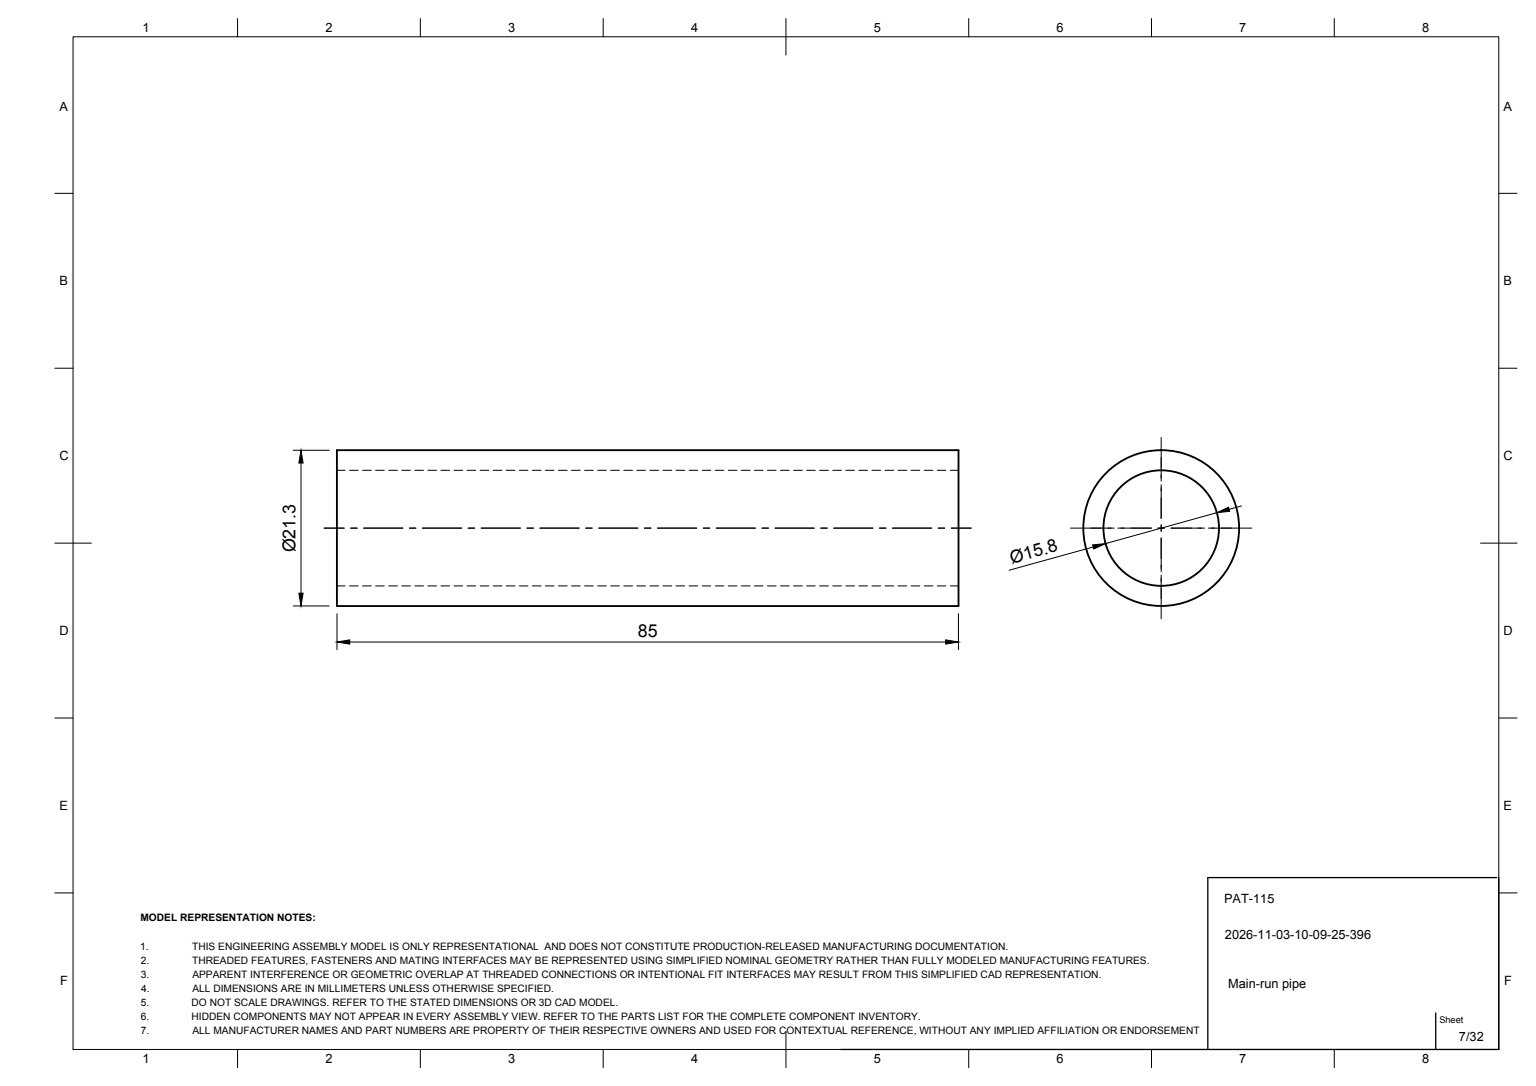
ISO-10303-21;
HEADER;
/* Generated by software containing ST-Developer
 * from STEP Tools, Inc. (www.steptools.com) 
 */

FILE_DESCRIPTION(
/* description */ ('Union bypass pipe loop'),
/* implementation_level */ '2;1');

FILE_NAME(
/* name */ 'Main-run pipe.step',
/* time_stamp */ '2026-10-27T21:00:29-07:00',
/* author */ (''),
/* organization */ (''),
/* preprocessor_version */ 'ST-DEVELOPER v20.2',
/* originating_system */ 'Autodesk Translation Framework v15.17.0.0',
/* authorisation */ '');

FILE_SCHEMA (('AUTOMOTIVE_DESIGN { 1 0 10303 214 3 1 1 }'));
ENDSEC;

DATA;
#10=MECHANICAL_DESIGN_GEOMETRIC_PRESENTATION_REPRESENTATION('',(#461),#10095);
#397=SHAPE_REPRESENTATION_RELATIONSHIP('SRR','None',#10266,#429);
#429=ADVANCED_BREP_SHAPE_REPRESENTATION('',(#491),#10078);
#461=STYLED_ITEM('',(#10486),#491);
#491=MANIFOLD_SOLID_BREP('Body1',#5534);
#582=FACE_BOUND('',#1413,.T.);
#583=FACE_BOUND('',#1415,.T.);
#732=PLANE('',#6291);
#733=PLANE('',#6292);
#1007=FACE_OUTER_BOUND('',#1410,.T.);
#1008=FACE_OUTER_BOUND('',#1411,.T.);
#1009=FACE_OUTER_BOUND('',#1412,.T.);
#1010=FACE_OUTER_BOUND('',#1414,.T.);
#1410=EDGE_LOOP('',(#4440,#4441,#4442,#4443));
#1411=EDGE_LOOP('',(#4444,#4445,#4446,#4447));
#1412=EDGE_LOOP('',(#4448));
#1413=EDGE_LOOP('',(#4449));
#1414=EDGE_LOOP('',(#4450));
#1415=EDGE_LOOP('',(#4451));
#1809=LINE('',#9257,#2185);
#1810=LINE('',#9263,#2186);
#2185=VECTOR('',#7569,0.79);
#2186=VECTOR('',#7576,1.065);
#2514=CIRCLE('',#6286,0.79);
#2515=CIRCLE('',#6287,0.79);
#2516=CIRCLE('',#6289,1.065);
#2517=CIRCLE('',#6290,1.065);
#2858=VERTEX_POINT('',#9254);
#2859=VERTEX_POINT('',#9256);
#2860=VERTEX_POINT('',#9260);
#2861=VERTEX_POINT('',#9262);
#3418=EDGE_CURVE('',#2858,#2858,#2514,.T.);
#3419=EDGE_CURVE('',#2858,#2859,#1809,.T.);
#3420=EDGE_CURVE('',#2859,#2859,#2515,.T.);
#3421=EDGE_CURVE('',#2860,#2860,#2516,.T.);
#3422=EDGE_CURVE('',#2860,#2861,#1810,.T.);
#3423=EDGE_CURVE('',#2861,#2861,#2517,.T.);
#4440=ORIENTED_EDGE('',*,*,#3418,.F.);
#4441=ORIENTED_EDGE('',*,*,#3419,.T.);
#4442=ORIENTED_EDGE('',*,*,#3420,.T.);
#4443=ORIENTED_EDGE('',*,*,#3419,.F.);
#4444=ORIENTED_EDGE('',*,*,#3421,.F.);
#4445=ORIENTED_EDGE('',*,*,#3422,.T.);
#4446=ORIENTED_EDGE('',*,*,#3423,.T.);
#4447=ORIENTED_EDGE('',*,*,#3422,.F.);
#4448=ORIENTED_EDGE('',*,*,#3421,.T.);
#4449=ORIENTED_EDGE('',*,*,#3418,.T.);
#4450=ORIENTED_EDGE('',*,*,#3423,.F.);
#4451=ORIENTED_EDGE('',*,*,#3420,.F.);
#5141=CYLINDRICAL_SURFACE('',#6285,0.79);
#5142=CYLINDRICAL_SURFACE('',#6288,1.065);
#5356=ADVANCED_FACE('',(#1007),#5141,.F.);
#5357=ADVANCED_FACE('',(#1008),#5142,.T.);
#5358=ADVANCED_FACE('',(#1009,#582),#732,.T.);
#5359=ADVANCED_FACE('',(#1010,#583),#733,.F.);
#5534=CLOSED_SHELL('',(#5356,#5357,#5358,#5359));
#6284=AXIS2_PLACEMENT_3D('',#9252,#7563,#7564);
#6285=AXIS2_PLACEMENT_3D('',#9253,#7565,#7566);
#6286=AXIS2_PLACEMENT_3D('',#9255,#7567,#7568);
#6287=AXIS2_PLACEMENT_3D('',#9258,#7570,#7571);
#6288=AXIS2_PLACEMENT_3D('',#9259,#7572,#7573);
#6289=AXIS2_PLACEMENT_3D('',#9261,#7574,#7575);
#6290=AXIS2_PLACEMENT_3D('',#9264,#7577,#7578);
#6291=AXIS2_PLACEMENT_3D('',#9265,#7579,#7580);
#6292=AXIS2_PLACEMENT_3D('',#9266,#7581,#7582);
#7563=DIRECTION('axis',(0.,0.,1.));
#7564=DIRECTION('refdir',(1.,0.,0.));
#7565=DIRECTION('center_axis',(1.,0.,0.));
#7566=DIRECTION('ref_axis',(0.,0.,-1.));
#7567=DIRECTION('center_axis',(-1.,0.,0.));
#7568=DIRECTION('ref_axis',(0.,0.,-1.));
#7569=DIRECTION('',(-1.,0.,0.));
#7570=DIRECTION('center_axis',(-1.,0.,0.));
#7571=DIRECTION('ref_axis',(0.,0.,-1.));
#7572=DIRECTION('center_axis',(1.,0.,0.));
#7573=DIRECTION('ref_axis',(0.,0.,-1.));
#7574=DIRECTION('center_axis',(1.,0.,0.));
#7575=DIRECTION('ref_axis',(0.,0.,-1.));
#7576=DIRECTION('',(-1.,0.,0.));
#7577=DIRECTION('center_axis',(1.,0.,0.));
#7578=DIRECTION('ref_axis',(0.,0.,-1.));
#7579=DIRECTION('center_axis',(1.,0.,0.));
#7580=DIRECTION('ref_axis',(0.,0.,-1.));
#7581=DIRECTION('center_axis',(1.,0.,0.));
#7582=DIRECTION('ref_axis',(0.,0.,-1.));
#9252=CARTESIAN_POINT('',(0.,0.,0.));
#9253=CARTESIAN_POINT('Origin',(-11.3,0.,5.));
#9254=CARTESIAN_POINT('',(-2.8,-9.67470971326409E-17,5.79));
#9255=CARTESIAN_POINT('Origin',(-2.8,0.,5.));
#9256=CARTESIAN_POINT('',(-11.3,-9.67470971326409E-17,5.79));
#9257=CARTESIAN_POINT('',(-11.3,-9.67470971326409E-17,5.79));
#9258=CARTESIAN_POINT('Origin',(-11.3,0.,5.));
#9259=CARTESIAN_POINT('Origin',(-11.3,0.,5.));
#9260=CARTESIAN_POINT('',(-2.8,-1.30424884109193E-16,6.065));
#9261=CARTESIAN_POINT('Origin',(-2.8,0.,5.));
#9262=CARTESIAN_POINT('',(-11.3,-1.30424884109193E-16,6.065));
#9263=CARTESIAN_POINT('',(-11.3,-1.30424884109193E-16,6.065));
#9264=CARTESIAN_POINT('Origin',(-11.3,0.,5.));
#9265=CARTESIAN_POINT('Origin',(-2.8,0.,5.));
#9266=CARTESIAN_POINT('Origin',(-11.3,0.,5.));
#10041=UNCERTAINTY_MEASURE_WITH_UNIT(LENGTH_MEASURE(0.001),#10096,
'DISTANCE_ACCURACY_VALUE',
'Maximum model space distance between geometric entities at asserted c
onnectivities');
#10058=UNCERTAINTY_MEASURE_WITH_UNIT(LENGTH_MEASURE(0.001),#10096,
'DISTANCE_ACCURACY_VALUE',
'Maximum model space distance between geometric entities at asserted c
onnectivities');
#10078=(
GEOMETRIC_REPRESENTATION_CONTEXT(3)
GLOBAL_UNCERTAINTY_ASSIGNED_CONTEXT((#10041))
GLOBAL_UNIT_ASSIGNED_CONTEXT((#10096,#10098,#10099))
REPRESENTATION_CONTEXT('','3D')
);
#10095=(
GEOMETRIC_REPRESENTATION_CONTEXT(3)
GLOBAL_UNCERTAINTY_ASSIGNED_CONTEXT((#10058))
GLOBAL_UNIT_ASSIGNED_CONTEXT((#10096,#10098,#10099))
REPRESENTATION_CONTEXT('','3D')
);
#10096=(
LENGTH_UNIT()
NAMED_UNIT(*)
SI_UNIT(.CENTI.,.METRE.)
);
#10098=(
NAMED_UNIT(*)
PLANE_ANGLE_UNIT()
SI_UNIT($,.RADIAN.)
);
#10099=(
NAMED_UNIT(*)
SI_UNIT($,.STERADIAN.)
SOLID_ANGLE_UNIT()
);
#10119=SHAPE_DEFINITION_REPRESENTATION(#10190,#10266);
#10190=PRODUCT_DEFINITION_SHAPE('',$,#10303);
#10266=SHAPE_REPRESENTATION('',(#6284),#10078);
#10283=PRODUCT_DEFINITION_CONTEXT('part definition',#10393,'design');
#10303=PRODUCT_DEFINITION('Main-run pipe','Main-run pipe',#10339,#10283);
#10339=PRODUCT_DEFINITION_FORMATION('',$,#10414);
#10393=APPLICATION_CONTEXT(
'Core Data for Automotive Mechanical Design Process');
#10394=PRODUCT_CONTEXT('part definition',#10393,'mechanical');
#10414=PRODUCT('Main-run pipe','Main-run pipe','Main-run pipe',(#10394));
#10480=COLOUR_RGB('Light Blue',0.38,0.62,0.78);
#10481=FILL_AREA_STYLE_COLOUR('',#10480);
#10482=FILL_AREA_STYLE('',(#10481));
#10483=SURFACE_STYLE_FILL_AREA(#10482);
#10484=SURFACE_SIDE_STYLE('',(#10483));
#10485=SURFACE_STYLE_USAGE(.BOTH.,#10484);
#10486=PRESENTATION_STYLE_ASSIGNMENT((#10485));
ENDSEC;
END-ISO-10303-21;
